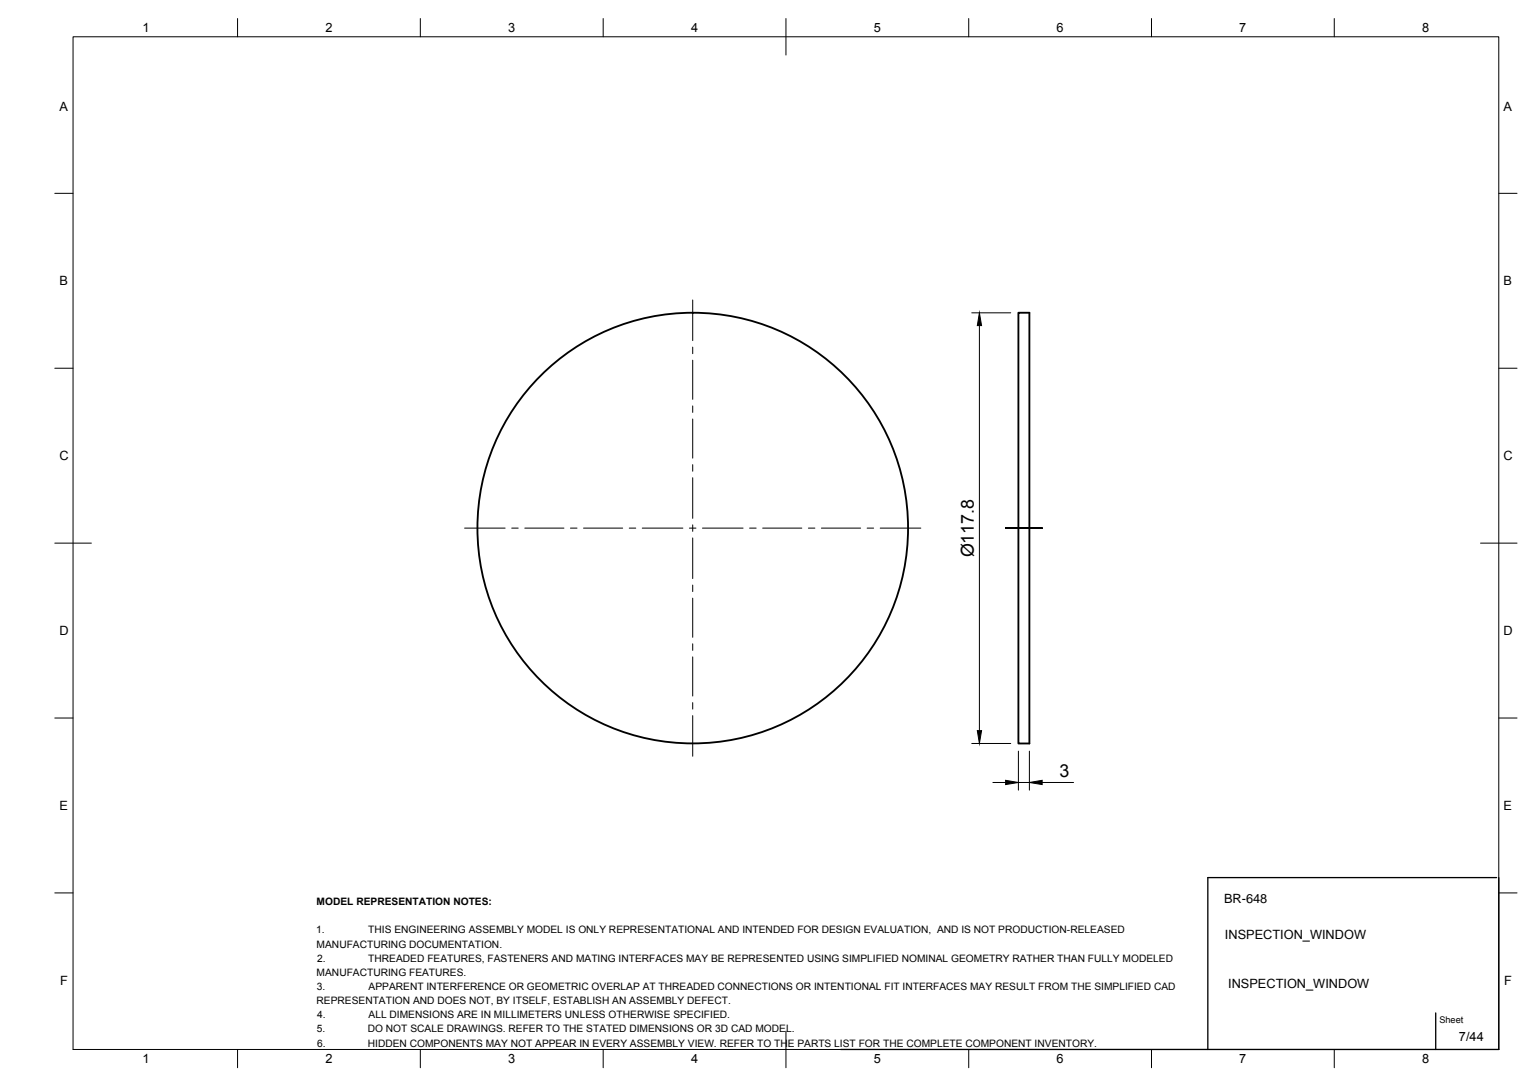
ISO-10303-21;
HEADER;
FILE_DESCRIPTION((''),'2;1');
FILE_NAME('INSPECTION_WINDOW.step','2026-10-01T22:05:39-07:00',(''),(''),'','','');
FILE_SCHEMA (('AUTOMOTIVE_DESIGN { 1 0 10303 214 3 1 1 }'));
ENDSEC;
DATA;
#10=MECHANICAL_DESIGN_GEOMETRIC_PRESENTATION_REPRESENTATION('',(#607),#24628);
#523=SHAPE_REPRESENTATION_RELATIONSHIP('SRR','None',#24795,#565) ;
#565=ADVANCED_BREP_SHAPE_REPRESENTATION('',(#649),#24585) ;
#607=STYLED_ITEM('',(#25032),#649) ;
#649=MANIFOLD_SOLID_BREP('INSPECTION_WINDOW',#13116) ;
#1062=LINE('',#20130,#1898) ;
#1898=VECTOR('',#15763,5.89) ;
#2708=CYLINDRICAL_SURFACE('',#13806,5.89) ;
#3014=FACE_OUTER_BOUND('',#3830,.T.) ;
#3015=FACE_OUTER_BOUND('',#3831,.T.) ;
#3016=FACE_OUTER_BOUND('',#3832,.T.) ;
#3830=EDGE_LOOP('',(#8793,#8794,#8795,#8796)) ;
#3831=EDGE_LOOP('',(#8797)) ;
#3832=EDGE_LOOP('',(#8798)) ;
#4838=CIRCLE('',#13807,5.89) ;
#4839=CIRCLE('',#13808,5.89) ;
#5639=VERTEX_POINT('',#20127) ;
#5640=VERTEX_POINT('',#20129) ;
#6886=EDGE_CURVE('',#5639,#5639,#4838,.T.) ;
#6887=EDGE_CURVE('',#5639,#5640,#1062,.T.) ;
#6888=EDGE_CURVE('',#5640,#5640,#4839,.T.) ;
#8793=ORIENTED_EDGE('',*,*,#6886,.F.) ;
#8794=ORIENTED_EDGE('',*,*,#6887,.T.) ;
#8795=ORIENTED_EDGE('',*,*,#6888,.F.) ;
#8796=ORIENTED_EDGE('',*,*,#6887,.F.) ;
#8797=ORIENTED_EDGE('',*,*,#6888,.T.) ;
#8798=ORIENTED_EDGE('',*,*,#6886,.T.) ;
#12022=PLANE('',#13809) ;
#12023=PLANE('',#13810) ;
#12409=ADVANCED_FACE('',(#3014),#2708,.T.) ;
#12410=ADVANCED_FACE('',(#3015),#12022,.T.) ;
#12411=ADVANCED_FACE('',(#3016),#12023,.T.) ;
#13116=CLOSED_SHELL('',(#12409,#12410,#12411)) ;
#13805=AXIS2_PLACEMENT_3D('',#20125,#15757,#15758) ;
#13806=AXIS2_PLACEMENT_3D('',#20126,#15759,#15760) ;
#13807=AXIS2_PLACEMENT_3D('',#20128,#15761,#15762) ;
#13808=AXIS2_PLACEMENT_3D('',#20131,#15764,#15765) ;
#13809=AXIS2_PLACEMENT_3D('',#20132,#15766,#15767) ;
#13810=AXIS2_PLACEMENT_3D('',#20133,#15768,#15769) ;
#15757=DIRECTION('axis',(0.,0.,1.)) ;
#15758=DIRECTION('refdir',(1.,0.,0.)) ;
#15759=DIRECTION('center_axis',(0.,1.,0.)) ;
#15760=DIRECTION('ref_axis',(1.,0.,0.)) ;
#15761=DIRECTION('center_axis',(0.,1.,0.)) ;
#15762=DIRECTION('ref_axis',(1.,0.,0.)) ;
#15763=DIRECTION('',(0.,-1.,0.)) ;
#15764=DIRECTION('center_axis',(0.,-1.,0.)) ;
#15765=DIRECTION('ref_axis',(1.,0.,0.)) ;
#15766=DIRECTION('center_axis',(0.,-1.,0.)) ;
#15767=DIRECTION('ref_axis',(-1.,0.,0.)) ;
#15768=DIRECTION('center_axis',(0.,1.,0.)) ;
#15769=DIRECTION('ref_axis',(1.,0.,0.)) ;
#20125=CARTESIAN_POINT('',(0.,0.,0.)) ;
#20126=CARTESIAN_POINT('Origin',(0.,3.85,0.)) ;
#20127=CARTESIAN_POINT('',(-5.89,4.,7.21316964697791E-16)) ;
#20128=CARTESIAN_POINT('Origin',(0.,4.,0.)) ;
#20129=CARTESIAN_POINT('',(-5.89,3.7,7.21316964697791E-16)) ;
#20130=CARTESIAN_POINT('',(-5.89,3.85,7.21316964697791E-16)) ;
#20131=CARTESIAN_POINT('Origin',(0.,3.7,0.)) ;
#20132=CARTESIAN_POINT('Origin',(0.,3.7,0.)) ;
#20133=CARTESIAN_POINT('Origin',(0.,4.,0.)) ;
#24537=UNCERTAINTY_MEASURE_WITH_UNIT(LENGTH_MEASURE(0.001),#24629,
'DISTANCE_ACCURACY_VALUE',
'Maximum model space distance between geometric entities at asserted c
onnectivities') ;
#24580=UNCERTAINTY_MEASURE_WITH_UNIT(LENGTH_MEASURE(0.001),#24629,
'DISTANCE_ACCURACY_VALUE',
'Maximum model space distance between geometric entities at asserted c
onnectivities') ;
#24585=(
GEOMETRIC_REPRESENTATION_CONTEXT(3)
GLOBAL_UNCERTAINTY_ASSIGNED_CONTEXT((#24537))
GLOBAL_UNIT_ASSIGNED_CONTEXT((#24629,#24631,#24632))
REPRESENTATION_CONTEXT('','3D')
) ;
#24628=(
GEOMETRIC_REPRESENTATION_CONTEXT(3)
GLOBAL_UNCERTAINTY_ASSIGNED_CONTEXT((#24580))
GLOBAL_UNIT_ASSIGNED_CONTEXT((#24629,#24631,#24632))
REPRESENTATION_CONTEXT('','3D')
) ;
#24629=(
LENGTH_UNIT()
NAMED_UNIT(*)
SI_UNIT(.CENTI.,.METRE.)
) ;
#24631=(
NAMED_UNIT(*)
PLANE_ANGLE_UNIT()
SI_UNIT($,.RADIAN.)
) ;
#24632=(
NAMED_UNIT(*)
SI_UNIT($,.STERADIAN.)
SOLID_ANGLE_UNIT()
) ;
#24637=SHAPE_DEFINITION_REPRESENTATION(#24684,#24795) ;
#24684=PRODUCT_DEFINITION_SHAPE('',$,#24843) ;
#24795=SHAPE_REPRESENTATION('',(#13805),#24585) ;
#24838=PRODUCT_DEFINITION_CONTEXT('part definition',#24981,'design') ;
#24843=PRODUCT_DEFINITION('INSPECTION_WINDOW','INSPECTION_WINDOW',
#24890,#24838) ;
#24890=PRODUCT_DEFINITION_FORMATION('',$,#24987) ;
#24981=APPLICATION_CONTEXT(
'Core Data for Automotive Mechanical Design Process') ;
#24982=PRODUCT_CONTEXT('part definition',#24981,'mechanical') ;
#24987=PRODUCT('INSPECTION_WINDOW','INSPECTION_WINDOW',$,(#24982)) ;
#25032=PRESENTATION_STYLE_ASSIGNMENT((#25042)) ;
#25042=SURFACE_STYLE_USAGE(.BOTH.,#25052) ;
#25052=SURFACE_SIDE_STYLE('',(#25062)) ;
#25062=SURFACE_STYLE_FILL_AREA(#25072) ;
#25072=FILL_AREA_STYLE('Plastic - Glossy (Grey)',(#25082)) ;
#25082=FILL_AREA_STYLE_COLOUR('Plastic - Glossy (Grey)',#25092) ;
#25092=COLOUR_RGB('Plastic - Glossy (Grey)', 0.08235294, 0.09019608, 0.10196078) ;
ENDSEC;
END-ISO-10303-21;
